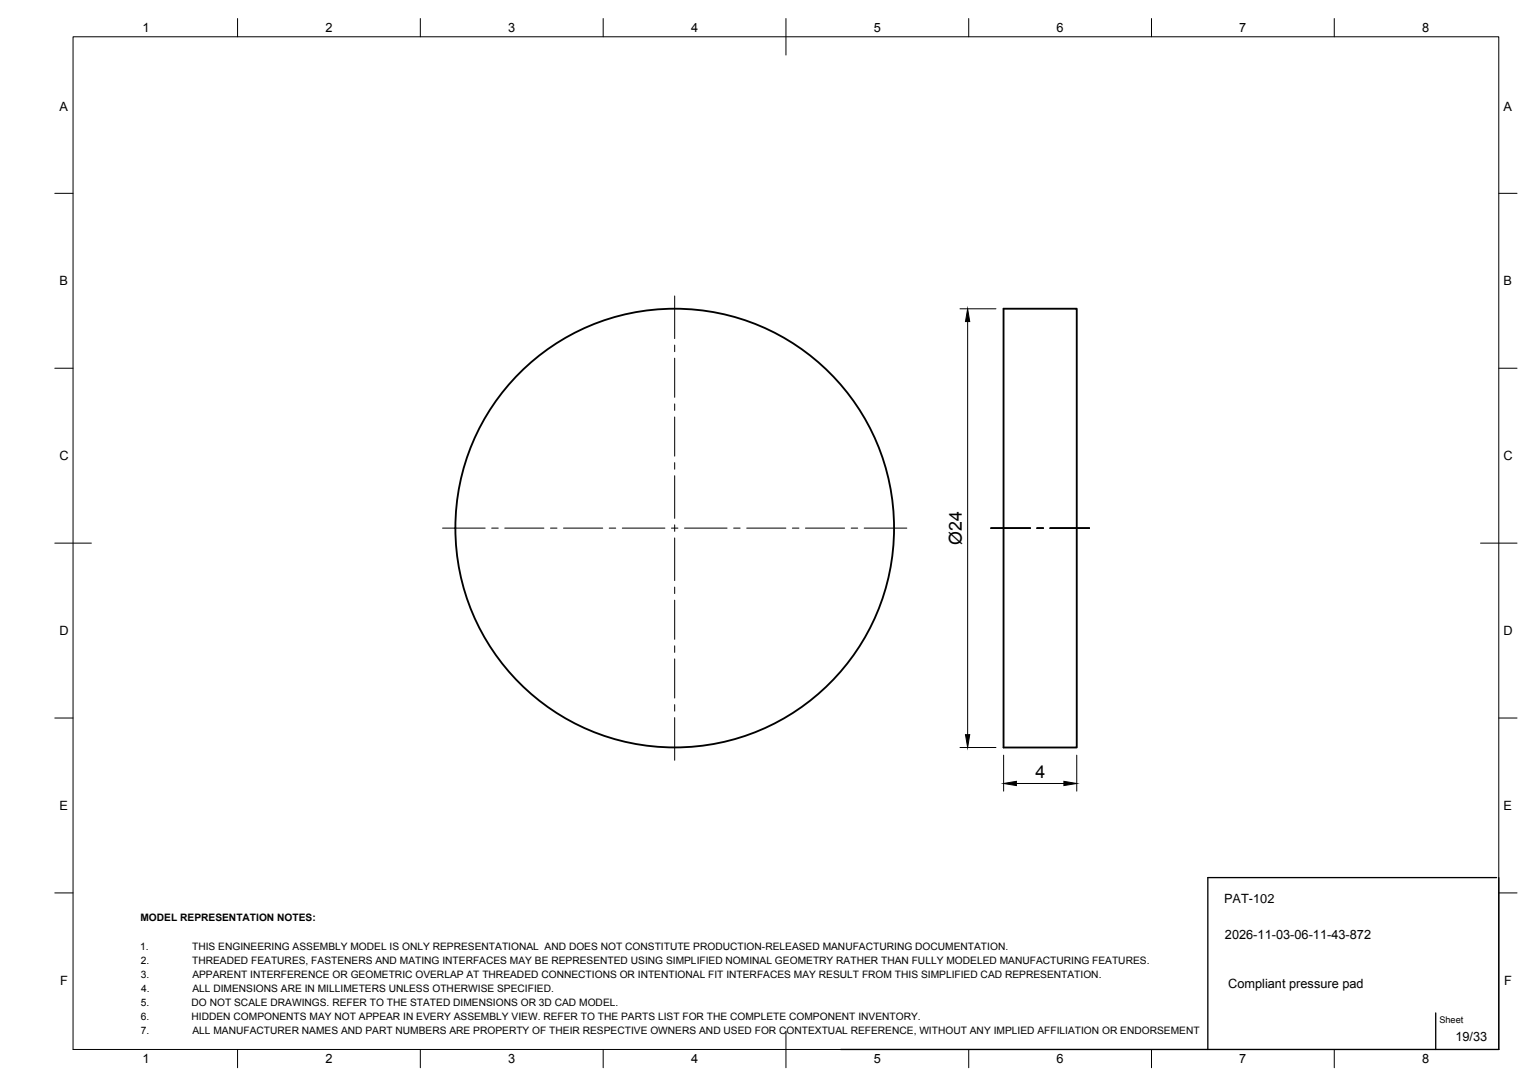
ISO-10303-21;
HEADER;
/* Generated by software containing ST-Developer
 * from STEP Tools, Inc. (www.steptools.com) 
 */

FILE_DESCRIPTION(
/* description */ ('Swing-away clamp arm'),
/* implementation_level */ '2;1');

FILE_NAME(
/* name */ 'Compliant pressure pad.step',
/* time_stamp */ '2026-10-28T03:26:03-07:00',
/* author */ (''),
/* organization */ (''),
/* preprocessor_version */ 'ST-DEVELOPER v20.2',
/* originating_system */ 'Autodesk Translation Framework v15.17.0.0',
/* authorisation */ '');

FILE_SCHEMA (('AUTOMOTIVE_DESIGN { 1 0 10303 214 3 1 1 }'));
ENDSEC;

DATA;
#10=MECHANICAL_DESIGN_GEOMETRIC_PRESENTATION_REPRESENTATION('',(#306),#10627);
#254=SHAPE_REPRESENTATION_RELATIONSHIP('SRR','None',#10753,#280);
#280=ADVANCED_BREP_SHAPE_REPRESENTATION('',(#339),#10612);
#306=STYLED_ITEM('',(#10958),#339);
#339=MANIFOLD_SOLID_BREP('Body1',#4913);
#576=PLANE('',#5577);
#577=PLANE('',#5578);
#820=FACE_OUTER_BOUND('',#1201,.T.);
#821=FACE_OUTER_BOUND('',#1202,.T.);
#822=FACE_OUTER_BOUND('',#1203,.T.);
#1201=EDGE_LOOP('',(#4035,#4036,#4037,#4038));
#1202=EDGE_LOOP('',(#4039));
#1203=EDGE_LOOP('',(#4040));
#1585=LINE('',#9667,#1907);
#1907=VECTOR('',#6810,1.2);
#2137=CIRCLE('',#5575,1.2);
#2138=CIRCLE('',#5576,1.2);
#2512=VERTEX_POINT('',#9664);
#2513=VERTEX_POINT('',#9666);
#3050=EDGE_CURVE('',#2512,#2512,#2137,.T.);
#3051=EDGE_CURVE('',#2512,#2513,#1585,.T.);
#3052=EDGE_CURVE('',#2513,#2513,#2138,.T.);
#4035=ORIENTED_EDGE('',*,*,#3050,.F.);
#4036=ORIENTED_EDGE('',*,*,#3051,.T.);
#4037=ORIENTED_EDGE('',*,*,#3052,.T.);
#4038=ORIENTED_EDGE('',*,*,#3051,.F.);
#4039=ORIENTED_EDGE('',*,*,#3050,.T.);
#4040=ORIENTED_EDGE('',*,*,#3052,.F.);
#4558=CYLINDRICAL_SURFACE('',#5574,1.2);
#4775=ADVANCED_FACE('',(#820),#4558,.T.);
#4776=ADVANCED_FACE('',(#821),#576,.T.);
#4777=ADVANCED_FACE('',(#822),#577,.F.);
#4913=CLOSED_SHELL('',(#4775,#4776,#4777));
#5573=AXIS2_PLACEMENT_3D('',#9662,#6804,#6805);
#5574=AXIS2_PLACEMENT_3D('',#9663,#6806,#6807);
#5575=AXIS2_PLACEMENT_3D('',#9665,#6808,#6809);
#5576=AXIS2_PLACEMENT_3D('',#9668,#6811,#6812);
#5577=AXIS2_PLACEMENT_3D('',#9669,#6813,#6814);
#5578=AXIS2_PLACEMENT_3D('',#9670,#6815,#6816);
#6804=DIRECTION('axis',(0.,0.,1.));
#6805=DIRECTION('refdir',(1.,0.,0.));
#6806=DIRECTION('center_axis',(0.,0.,1.));
#6807=DIRECTION('ref_axis',(1.,0.,0.));
#6808=DIRECTION('center_axis',(0.,0.,1.));
#6809=DIRECTION('ref_axis',(1.,0.,0.));
#6810=DIRECTION('',(0.,0.,-1.));
#6811=DIRECTION('center_axis',(0.,0.,1.));
#6812=DIRECTION('ref_axis',(1.,0.,0.));
#6813=DIRECTION('center_axis',(0.,0.,1.));
#6814=DIRECTION('ref_axis',(1.,0.,0.));
#6815=DIRECTION('center_axis',(0.,0.,1.));
#6816=DIRECTION('ref_axis',(1.,0.,0.));
#9662=CARTESIAN_POINT('',(0.,0.,0.));
#9663=CARTESIAN_POINT('Origin',(12.,0.,6.));
#9664=CARTESIAN_POINT('',(10.8,-1.46957615897682E-16,6.4));
#9665=CARTESIAN_POINT('Origin',(12.,0.,6.4));
#9666=CARTESIAN_POINT('',(10.8,-1.46957615897682E-16,6.));
#9667=CARTESIAN_POINT('',(10.8,-1.46957615897682E-16,6.));
#9668=CARTESIAN_POINT('Origin',(12.,0.,6.));
#9669=CARTESIAN_POINT('Origin',(12.,0.,6.4));
#9670=CARTESIAN_POINT('Origin',(12.,0.,6.));
#10580=UNCERTAINTY_MEASURE_WITH_UNIT(LENGTH_MEASURE(0.001),#10628,
'DISTANCE_ACCURACY_VALUE',
'Maximum model space distance between geometric entities at asserted c
onnectivities');
#10595=UNCERTAINTY_MEASURE_WITH_UNIT(LENGTH_MEASURE(0.001),#10628,
'DISTANCE_ACCURACY_VALUE',
'Maximum model space distance between geometric entities at asserted c
onnectivities');
#10612=(
GEOMETRIC_REPRESENTATION_CONTEXT(3)
GLOBAL_UNCERTAINTY_ASSIGNED_CONTEXT((#10580))
GLOBAL_UNIT_ASSIGNED_CONTEXT((#10628,#10630,#10631))
REPRESENTATION_CONTEXT('','3D')
);
#10627=(
GEOMETRIC_REPRESENTATION_CONTEXT(3)
GLOBAL_UNCERTAINTY_ASSIGNED_CONTEXT((#10595))
GLOBAL_UNIT_ASSIGNED_CONTEXT((#10628,#10630,#10631))
REPRESENTATION_CONTEXT('','3D')
);
#10628=(
LENGTH_UNIT()
NAMED_UNIT(*)
SI_UNIT(.CENTI.,.METRE.)
);
#10630=(
NAMED_UNIT(*)
PLANE_ANGLE_UNIT()
SI_UNIT($,.RADIAN.)
);
#10631=(
NAMED_UNIT(*)
SI_UNIT($,.STERADIAN.)
SOLID_ANGLE_UNIT()
);
#10648=SHAPE_DEFINITION_REPRESENTATION(#10689,#10753);
#10689=PRODUCT_DEFINITION_SHAPE('',$,#10785);
#10753=SHAPE_REPRESENTATION('',(#5573),#10612);
#10768=PRODUCT_DEFINITION_CONTEXT('part definition',#10863,'design');
#10785=PRODUCT_DEFINITION('Compliant pressure pad',
'Compliant pressure pad',#10816,#10768);
#10816=PRODUCT_DEFINITION_FORMATION('',$,#10881);
#10863=APPLICATION_CONTEXT(
'Core Data for Automotive Mechanical Design Process');
#10864=PRODUCT_CONTEXT('part definition',#10863,'mechanical');
#10881=PRODUCT('Compliant pressure pad','Compliant pressure pad',
'Compliant pressure pad',(#10864));
#10952=COLOUR_RGB('Sky Blue',0.24,0.69,0.87);
#10953=FILL_AREA_STYLE_COLOUR('',#10952);
#10954=FILL_AREA_STYLE('',(#10953));
#10955=SURFACE_STYLE_FILL_AREA(#10954);
#10956=SURFACE_SIDE_STYLE('',(#10955));
#10957=SURFACE_STYLE_USAGE(.BOTH.,#10956);
#10958=PRESENTATION_STYLE_ASSIGNMENT((#10957));
ENDSEC;
END-ISO-10303-21;
